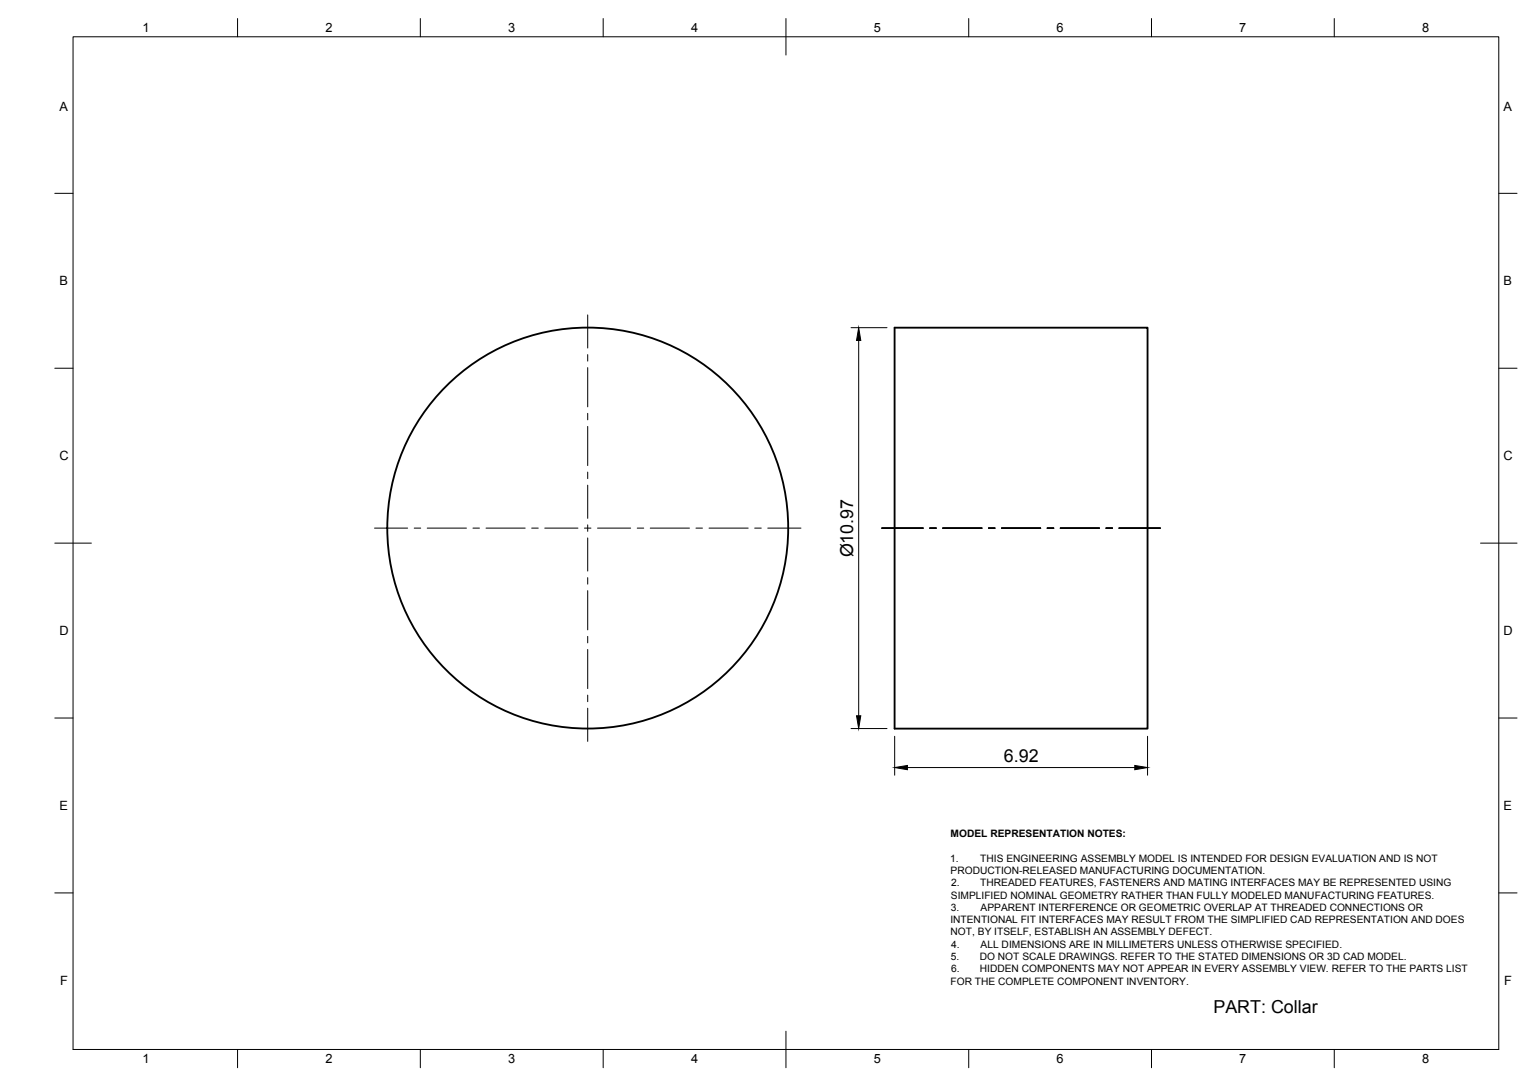
ISO-10303-21;
HEADER;
/* Generated by software containing ST-Developer
 * from STEP Tools, Inc. (www.steptools.com) 
 */

FILE_DESCRIPTION(
/* description */ (''),
/* implementation_level */ '2;1');

FILE_NAME(
/* name */ 'Collar.step',
/* time_stamp */ '2026-10-05T01:33:24-07:00',
/* author */ (''),
/* organization */ (''),
/* preprocessor_version */ 'ST-DEVELOPER v20.2',
/* originating_system */ 'Autodesk Translation Framework v15.15.0.0',
/* authorisation */ '');

FILE_SCHEMA (('AUTOMOTIVE_DESIGN { 1 0 10303 214 3 1 1 }'));
ENDSEC;

DATA;
#10=MECHANICAL_DESIGN_GEOMETRIC_PRESENTATION_REPRESENTATION('',(#91),#1128);
#71=SHAPE_REPRESENTATION_RELATIONSHIP('SRR','None',#1175,#81);
#81=ADVANCED_BREP_SHAPE_REPRESENTATION('',(#101),#1127);
#91=STYLED_ITEM('',(#1225),#101);
#101=MANIFOLD_SOLID_BREP('Body1',#530);
#118=LINE('',#1094,#135);
#135=VECTOR('',#935,5.48257260644808);
#145=CYLINDRICAL_SURFACE('',#730,5.48257260644808);
#184=FACE_OUTER_BOUND('',#225,.T.);
#185=FACE_OUTER_BOUND('',#226,.T.);
#186=FACE_OUTER_BOUND('',#227,.T.);
#225=EDGE_LOOP('',(#454));
#226=EDGE_LOOP('',(#455));
#227=EDGE_LOOP('',(#456,#457,#458,#459));
#263=CIRCLE('',#727,5.48257260644808);
#264=CIRCLE('',#729,5.48257260644808);
#296=VERTEX_POINT('',#1088);
#297=VERTEX_POINT('',#1091);
#349=EDGE_CURVE('',#296,#296,#263,.T.);
#350=EDGE_CURVE('',#297,#297,#264,.T.);
#351=EDGE_CURVE('',#296,#297,#118,.T.);
#454=ORIENTED_EDGE('',*,*,#349,.T.);
#455=ORIENTED_EDGE('',*,*,#350,.F.);
#456=ORIENTED_EDGE('',*,*,#349,.F.);
#457=ORIENTED_EDGE('',*,*,#351,.T.);
#458=ORIENTED_EDGE('',*,*,#350,.T.);
#459=ORIENTED_EDGE('',*,*,#351,.F.);
#478=PLANE('',#726);
#479=PLANE('',#728);
#518=ADVANCED_FACE('',(#184),#478,.T.);
#519=ADVANCED_FACE('',(#185),#479,.T.);
#520=ADVANCED_FACE('',(#186),#145,.T.);
#530=CLOSED_SHELL('',(#518,#519,#520));
#725=AXIS2_PLACEMENT_3D('',#1086,#923,#924);
#726=AXIS2_PLACEMENT_3D('',#1087,#925,#926);
#727=AXIS2_PLACEMENT_3D('',#1089,#927,#928);
#728=AXIS2_PLACEMENT_3D('',#1090,#929,#930);
#729=AXIS2_PLACEMENT_3D('',#1092,#931,#932);
#730=AXIS2_PLACEMENT_3D('',#1093,#933,#934);
#923=DIRECTION('axis',(0.,0.,1.));
#924=DIRECTION('refdir',(1.,0.,0.));
#925=DIRECTION('center_axis',(1.,0.,0.));
#926=DIRECTION('ref_axis',(0.,0.,-1.));
#927=DIRECTION('center_axis',(1.,0.,0.));
#928=DIRECTION('ref_axis',(0.,0.,-1.));
#929=DIRECTION('center_axis',(-1.,0.,0.));
#930=DIRECTION('ref_axis',(0.,0.,1.));
#931=DIRECTION('center_axis',(1.,0.,0.));
#932=DIRECTION('ref_axis',(0.,0.,-1.));
#933=DIRECTION('center_axis',(1.,0.,0.));
#934=DIRECTION('ref_axis',(0.,0.,-1.));
#935=DIRECTION('',(-1.,0.,0.));
#1086=CARTESIAN_POINT('',(0.,0.,0.));
#1087=CARTESIAN_POINT('Origin',(47.3085747246001,0.,0.));
#1088=CARTESIAN_POINT('',(47.3085747246001,-6.71421499357961E-16,5.48257260644808));
#1089=CARTESIAN_POINT('Origin',(47.3085747246001,0.,0.));
#1090=CARTESIAN_POINT('Origin',(40.3908939752244,0.,-5.48257260644808));
#1091=CARTESIAN_POINT('',(40.3908939752244,-6.71421499357961E-16,5.48257260644808));
#1092=CARTESIAN_POINT('Origin',(40.3908939752244,0.,0.));
#1093=CARTESIAN_POINT('Origin',(43.8497343499122,0.,0.));
#1094=CARTESIAN_POINT('',(43.8497343499122,-6.7142149935796E-16,5.48257260644808));
#1115=UNCERTAINTY_MEASURE_WITH_UNIT(LENGTH_MEASURE(0.01),#1129,
'DISTANCE_ACCURACY_VALUE',
'Maximum model space distance between geometric entities at asserted c
onnectivities');
#1116=UNCERTAINTY_MEASURE_WITH_UNIT(LENGTH_MEASURE(0.01),#1129,
'DISTANCE_ACCURACY_VALUE',
'Maximum model space distance between geometric entities at asserted c
onnectivities');
#1127=(
GEOMETRIC_REPRESENTATION_CONTEXT(3)
GLOBAL_UNCERTAINTY_ASSIGNED_CONTEXT((#1115))
GLOBAL_UNIT_ASSIGNED_CONTEXT((#1129,#1131,#1132))
REPRESENTATION_CONTEXT('','3D')
);
#1128=(
GEOMETRIC_REPRESENTATION_CONTEXT(3)
GLOBAL_UNCERTAINTY_ASSIGNED_CONTEXT((#1116))
GLOBAL_UNIT_ASSIGNED_CONTEXT((#1129,#1131,#1132))
REPRESENTATION_CONTEXT('','3D')
);
#1129=(
LENGTH_UNIT()
NAMED_UNIT(*)
SI_UNIT(.MILLI.,.METRE.)
);
#1131=(
NAMED_UNIT(*)
PLANE_ANGLE_UNIT()
SI_UNIT($,.RADIAN.)
);
#1132=(
NAMED_UNIT(*)
SI_UNIT($,.STERADIAN.)
SOLID_ANGLE_UNIT()
);
#1143=SHAPE_DEFINITION_REPRESENTATION(#1154,#1175);
#1154=PRODUCT_DEFINITION_SHAPE('',$,#1187);
#1175=SHAPE_REPRESENTATION('',(#725),#1127);
#1176=PRODUCT_DEFINITION_CONTEXT('part definition',#1211,'design');
#1187=PRODUCT_DEFINITION('Collar','Collar',#1198,#1176);
#1198=PRODUCT_DEFINITION_FORMATION('',$,#1223);
#1211=APPLICATION_CONTEXT(
'Core Data for Automotive Mechanical Design Process');
#1212=PRODUCT_CONTEXT('part definition',#1211,'mechanical');
#1223=PRODUCT('Collar','Collar',$,(#1212));
#1225=PRESENTATION_STYLE_ASSIGNMENT((#1229));
#1229=SURFACE_STYLE_USAGE(.BOTH.,#1233);
#1233=SURFACE_SIDE_STYLE('',(#1237));
#1237=SURFACE_STYLE_FILL_AREA(#1241);
#1241=FILL_AREA_STYLE('Opaque(201,201,201)',(#1245));
#1245=FILL_AREA_STYLE_COLOUR('Opaque(201,201,201)',#1249);
#1249=COLOUR_RGB('Opaque(201,201,201)', 0.09019608, 0.27058824, 0.51372549);
ENDSEC;
END-ISO-10303-21;
